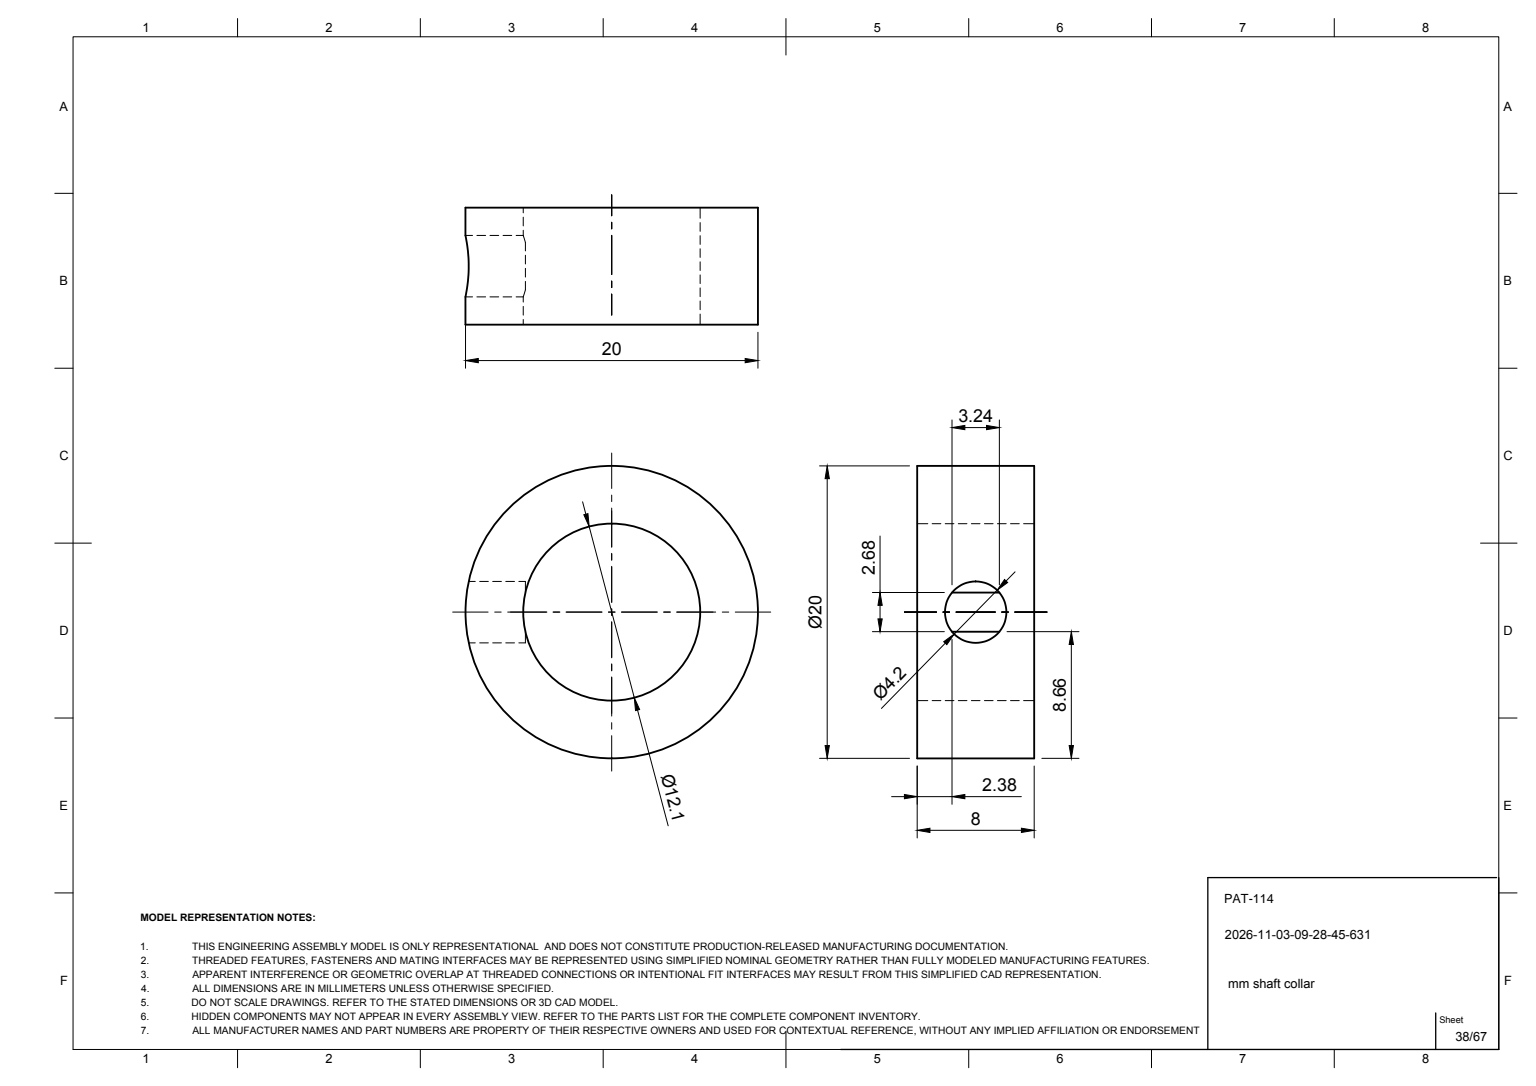
ISO-10303-21;
HEADER;
/* Generated by software containing ST-Developer
 * from STEP Tools, Inc. (www.steptools.com) 
 */

FILE_DESCRIPTION(
/* description */ ('Two-stage gear reducer in split housing'),
/* implementation_level */ '2;1');

FILE_NAME(
/* name */ 'mm shaft collar.step',
/* time_stamp */ '2026-10-28T03:22:31-07:00',
/* author */ (''),
/* organization */ (''),
/* preprocessor_version */ 'ST-DEVELOPER v20.2',
/* originating_system */ 'Autodesk Translation Framework v15.17.0.0',
/* authorisation */ '');

FILE_SCHEMA (('AUTOMOTIVE_DESIGN { 1 0 10303 214 3 1 1 }'));
ENDSEC;

DATA;
#10=MECHANICAL_DESIGN_GEOMETRIC_PRESENTATION_REPRESENTATION('',(#1278),#73366);
#963=B_SPLINE_CURVE_WITH_KNOTS('',3,(#25465,#25466,#25467,#25468,#25469,
#25470,#25471,#25472,#25473,#25474),.UNSPECIFIED.,.F.,.F.,(4,2,2,2,4),(0.818088904349178,
0.878131747417165,0.957937926194036,1.03774410497091,1.09778694803889),
 .UNSPECIFIED.);
#964=B_SPLINE_CURVE_WITH_KNOTS('',3,(#25480,#25481,#25482,#25483,#25484,
#25485,#25486,#25487,#25488,#25489,#25490,#25491,#25492,#25493,#25494,#25495,
#25496,#25497),.UNSPECIFIED.,.F.,.F.,(4,2,2,2,2,2,2,2,4),(0.,0.0793616477694788,
0.158723295538958,0.238079516586307,0.317435737633657,0.396791958681006,
0.476148179728356,0.555509827497835,0.634871475267313),.UNSPECIFIED.);
#965=B_SPLINE_CURVE_WITH_KNOTS('',3,(#25498,#25499,#25500,#25501,#25502,
#25503,#25504,#25505,#25506,#25507,#25508,#25509,#25510,#25511,#25512,#25513,
#25514,#25515),.UNSPECIFIED.,.F.,.F.,(4,2,2,2,2,2,2,2,4),(0.634871475267313,
0.714233123036792,0.793594770806271,0.87295099185362,0.95230721290097,1.03166343394832,
1.11101965499567,1.19038130276515,1.26974295053463),.UNSPECIFIED.);
#966=B_SPLINE_CURVE_WITH_KNOTS('',3,(#25518,#25519,#25520,#25521,#25522,
#25523,#25524,#25525,#25526,#25527),.UNSPECIFIED.,.F.,.F.,(4,2,2,2,4),(0.17946362021982,
0.239506463287808,0.319312642064679,0.39911882084155,0.459161663909537),
 .UNSPECIFIED.);
#1151=SHAPE_REPRESENTATION_RELATIONSHIP('SRR','None',#73641,#1207);
#1207=ADVANCED_BREP_SHAPE_REPRESENTATION('',(#1347),#73337);
#1278=STYLED_ITEM('',(#73988),#1347);
#1347=MANIFOLD_SOLID_BREP('Body1',#16168);
#1539=FACE_BOUND('',#3506,.T.);
#1540=FACE_BOUND('',#3508,.T.);
#1541=FACE_BOUND('',#3510,.T.);
#1542=FACE_BOUND('',#3512,.T.);
#1806=PLANE('',#17779);
#1807=PLANE('',#17784);
#1808=PLANE('',#17791);
#1809=PLANE('',#17792);
#2424=FACE_OUTER_BOUND('',#3502,.T.);
#2425=FACE_OUTER_BOUND('',#3503,.T.);
#2426=FACE_OUTER_BOUND('',#3504,.T.);
#2427=FACE_OUTER_BOUND('',#3505,.T.);
#2428=FACE_OUTER_BOUND('',#3507,.T.);
#2429=FACE_OUTER_BOUND('',#3509,.T.);
#2430=FACE_OUTER_BOUND('',#3511,.T.);
#3502=EDGE_LOOP('',(#12319,#12320));
#3503=EDGE_LOOP('',(#12321,#12322,#12323,#12324,#12325,#12326,#12327,#12328,
#12329));
#3504=EDGE_LOOP('',(#12330,#12331,#12332));
#3505=EDGE_LOOP('',(#12333,#12334,#12335,#12336));
#3506=EDGE_LOOP('',(#12337,#12338,#12339,#12340));
#3507=EDGE_LOOP('',(#12341,#12342,#12343,#12344));
#3508=EDGE_LOOP('',(#12345,#12346));
#3509=EDGE_LOOP('',(#12347));
#3510=EDGE_LOOP('',(#12348));
#3511=EDGE_LOOP('',(#12349));
#3512=EDGE_LOOP('',(#12350));
#4490=LINE('',#25461,#5514);
#4491=LINE('',#25478,#5515);
#4492=LINE('',#25529,#5516);
#4493=LINE('',#25534,#5517);
#4494=LINE('',#25540,#5518);
#5514=VECTOR('',#20828,1.);
#5515=VECTOR('',#20835,0.21);
#5516=VECTOR('',#20840,1.);
#5517=VECTOR('',#20845,0.605);
#5518=VECTOR('',#20852,1.);
#6544=CIRCLE('',#17780,0.21);
#6545=CIRCLE('',#17782,0.21);
#6546=CIRCLE('',#17783,0.21);
#6547=CIRCLE('',#17786,0.605);
#6548=CIRCLE('',#17787,0.605);
#6549=CIRCLE('',#17789,1.);
#6550=CIRCLE('',#17790,1.);
#7443=VERTEX_POINT('',#25459);
#7444=VERTEX_POINT('',#25460);
#7445=VERTEX_POINT('',#25464);
#7446=VERTEX_POINT('',#25475);
#7447=VERTEX_POINT('',#25477);
#7448=VERTEX_POINT('',#25479);
#7449=VERTEX_POINT('',#25516);
#7450=VERTEX_POINT('',#25531);
#7451=VERTEX_POINT('',#25533);
#7452=VERTEX_POINT('',#25537);
#7453=VERTEX_POINT('',#25539);
#9213=EDGE_CURVE('',#7443,#7444,#4490,.T.);
#9214=EDGE_CURVE('',#7443,#7444,#6544,.T.);
#9215=EDGE_CURVE('',#7445,#7443,#963,.T.);
#9216=EDGE_CURVE('',#7446,#7445,#6545,.T.);
#9217=EDGE_CURVE('',#7446,#7447,#4491,.T.);
#9218=EDGE_CURVE('',#7448,#7447,#964,.T.);
#9219=EDGE_CURVE('',#7447,#7448,#965,.T.);
#9220=EDGE_CURVE('',#7449,#7446,#6546,.T.);
#9221=EDGE_CURVE('',#7444,#7449,#966,.T.);
#9222=EDGE_CURVE('',#7449,#7445,#4492,.T.);
#9223=EDGE_CURVE('',#7450,#7450,#6547,.T.);
#9224=EDGE_CURVE('',#7450,#7451,#4493,.T.);
#9225=EDGE_CURVE('',#7451,#7451,#6548,.T.);
#9226=EDGE_CURVE('',#7452,#7452,#6549,.T.);
#9227=EDGE_CURVE('',#7452,#7453,#4494,.T.);
#9228=EDGE_CURVE('',#7453,#7453,#6550,.T.);
#12319=ORIENTED_EDGE('',*,*,#9213,.F.);
#12320=ORIENTED_EDGE('',*,*,#9214,.T.);
#12321=ORIENTED_EDGE('',*,*,#9215,.F.);
#12322=ORIENTED_EDGE('',*,*,#9216,.F.);
#12323=ORIENTED_EDGE('',*,*,#9217,.T.);
#12324=ORIENTED_EDGE('',*,*,#9218,.F.);
#12325=ORIENTED_EDGE('',*,*,#9219,.F.);
#12326=ORIENTED_EDGE('',*,*,#9217,.F.);
#12327=ORIENTED_EDGE('',*,*,#9220,.F.);
#12328=ORIENTED_EDGE('',*,*,#9221,.F.);
#12329=ORIENTED_EDGE('',*,*,#9214,.F.);
#12330=ORIENTED_EDGE('',*,*,#9222,.F.);
#12331=ORIENTED_EDGE('',*,*,#9220,.T.);
#12332=ORIENTED_EDGE('',*,*,#9216,.T.);
#12333=ORIENTED_EDGE('',*,*,#9223,.F.);
#12334=ORIENTED_EDGE('',*,*,#9224,.T.);
#12335=ORIENTED_EDGE('',*,*,#9225,.T.);
#12336=ORIENTED_EDGE('',*,*,#9224,.F.);
#12337=ORIENTED_EDGE('',*,*,#9221,.T.);
#12338=ORIENTED_EDGE('',*,*,#9222,.T.);
#12339=ORIENTED_EDGE('',*,*,#9215,.T.);
#12340=ORIENTED_EDGE('',*,*,#9213,.T.);
#12341=ORIENTED_EDGE('',*,*,#9226,.F.);
#12342=ORIENTED_EDGE('',*,*,#9227,.T.);
#12343=ORIENTED_EDGE('',*,*,#9228,.T.);
#12344=ORIENTED_EDGE('',*,*,#9227,.F.);
#12345=ORIENTED_EDGE('',*,*,#9218,.T.);
#12346=ORIENTED_EDGE('',*,*,#9219,.T.);
#12347=ORIENTED_EDGE('',*,*,#9226,.T.);
#12348=ORIENTED_EDGE('',*,*,#9223,.T.);
#12349=ORIENTED_EDGE('',*,*,#9228,.F.);
#12350=ORIENTED_EDGE('',*,*,#9225,.F.);
#15076=CYLINDRICAL_SURFACE('',#17781,0.21);
#15077=CYLINDRICAL_SURFACE('',#17785,0.605);
#15078=CYLINDRICAL_SURFACE('',#17788,1.);
#15631=ADVANCED_FACE('',(#2424),#1806,.T.);
#15632=ADVANCED_FACE('',(#2425),#15076,.F.);
#15633=ADVANCED_FACE('',(#2426),#1807,.T.);
#15634=ADVANCED_FACE('',(#2427,#1539),#15077,.F.);
#15635=ADVANCED_FACE('',(#2428,#1540),#15078,.T.);
#15636=ADVANCED_FACE('',(#2429,#1541),#1808,.T.);
#15637=ADVANCED_FACE('',(#2430,#1542),#1809,.F.);
#16168=CLOSED_SHELL('',(#15631,#15632,#15633,#15634,#15635,#15636,#15637));
#17778=AXIS2_PLACEMENT_3D('',#25457,#20824,#20825);
#17779=AXIS2_PLACEMENT_3D('',#25458,#20826,#20827);
#17780=AXIS2_PLACEMENT_3D('',#25462,#20829,#20830);
#17781=AXIS2_PLACEMENT_3D('',#25463,#20831,#20832);
#17782=AXIS2_PLACEMENT_3D('',#25476,#20833,#20834);
#17783=AXIS2_PLACEMENT_3D('',#25517,#20836,#20837);
#17784=AXIS2_PLACEMENT_3D('',#25528,#20838,#20839);
#17785=AXIS2_PLACEMENT_3D('',#25530,#20841,#20842);
#17786=AXIS2_PLACEMENT_3D('',#25532,#20843,#20844);
#17787=AXIS2_PLACEMENT_3D('',#25535,#20846,#20847);
#17788=AXIS2_PLACEMENT_3D('',#25536,#20848,#20849);
#17789=AXIS2_PLACEMENT_3D('',#25538,#20850,#20851);
#17790=AXIS2_PLACEMENT_3D('',#25541,#20853,#20854);
#17791=AXIS2_PLACEMENT_3D('',#25542,#20855,#20856);
#17792=AXIS2_PLACEMENT_3D('',#25543,#20857,#20858);
#20824=DIRECTION('axis',(0.,0.,1.));
#20825=DIRECTION('refdir',(1.,0.,0.));
#20826=DIRECTION('center_axis',(0.,0.,1.));
#20827=DIRECTION('ref_axis',(1.,0.,0.));
#20828=DIRECTION('',(0.,1.,0.));
#20829=DIRECTION('center_axis',(0.,0.,1.));
#20830=DIRECTION('ref_axis',(1.,0.,0.));
#20831=DIRECTION('center_axis',(0.,0.,1.));
#20832=DIRECTION('ref_axis',(1.,0.,0.));
#20833=DIRECTION('center_axis',(0.,0.,1.));
#20834=DIRECTION('ref_axis',(1.,0.,0.));
#20835=DIRECTION('',(0.,0.,1.));
#20836=DIRECTION('center_axis',(0.,0.,1.));
#20837=DIRECTION('ref_axis',(1.,0.,0.));
#20838=DIRECTION('center_axis',(0.,0.,1.));
#20839=DIRECTION('ref_axis',(1.,0.,0.));
#20840=DIRECTION('',(0.,-1.,0.));
#20841=DIRECTION('center_axis',(0.,1.,0.));
#20842=DIRECTION('ref_axis',(1.,0.,0.));
#20843=DIRECTION('center_axis',(0.,-1.,0.));
#20844=DIRECTION('ref_axis',(1.,0.,0.));
#20845=DIRECTION('',(0.,-1.,0.));
#20846=DIRECTION('center_axis',(0.,-1.,0.));
#20847=DIRECTION('ref_axis',(1.,0.,0.));
#20848=DIRECTION('center_axis',(0.,1.,0.));
#20849=DIRECTION('ref_axis',(1.,0.,0.));
#20850=DIRECTION('center_axis',(0.,1.,0.));
#20851=DIRECTION('ref_axis',(1.,0.,0.));
#20852=DIRECTION('',(0.,-1.,0.));
#20853=DIRECTION('center_axis',(0.,1.,0.));
#20854=DIRECTION('ref_axis',(1.,0.,0.));
#20855=DIRECTION('center_axis',(0.,1.,0.));
#20856=DIRECTION('ref_axis',(1.,0.,0.));
#20857=DIRECTION('center_axis',(0.,1.,0.));
#20858=DIRECTION('ref_axis',(1.,0.,0.));
#25457=CARTESIAN_POINT('',(0.,0.,0.));
#25458=CARTESIAN_POINT('Origin',(0.,-8.2,10.59));
#25459=CARTESIAN_POINT('',(0.133884278389952,-8.36178689687364,10.59));
#25460=CARTESIAN_POINT('',(0.133884278389952,-8.03821310312636,10.59));
#25461=CARTESIAN_POINT('',(0.133884278389952,-8.6,10.59));
#25462=CARTESIAN_POINT('Origin',(0.,-8.2,10.59));
#25463=CARTESIAN_POINT('Origin',(0.,-8.2,10.59));
#25464=CARTESIAN_POINT('',(-0.133884278389952,-8.36178689687364,10.59));
#25465=CARTESIAN_POINT('Ctrl Pts',(-0.133884278389951,-8.36178689687364,
10.59));
#25466=CARTESIAN_POINT('Ctrl Pts',(-0.118254395260798,-8.37472116821763,
10.5935467722442));
#25467=CARTESIAN_POINT('Ctrl Pts',(-0.100109787682296,-8.38579931658744,
10.5969822478996));
#25468=CARTESIAN_POINT('Ctrl Pts',(-0.0548298721325181,-8.40463856105443,
10.6030741628997));
#25469=CARTESIAN_POINT('Ctrl Pts',(-0.0266020595922904,-8.41,10.605));
#25470=CARTESIAN_POINT('Ctrl Pts',(0.0266020595922903,-8.41,10.605));
#25471=CARTESIAN_POINT('Ctrl Pts',(0.0548298721325192,-8.40463856105443,
10.6030741628997));
#25472=CARTESIAN_POINT('Ctrl Pts',(0.100109787682297,-8.38579931658744,
10.5969822478996));
#25473=CARTESIAN_POINT('Ctrl Pts',(0.118254395260798,-8.37472116821763,
10.5935467722442));
#25474=CARTESIAN_POINT('Ctrl Pts',(0.133884278389951,-8.36178689687364,
10.59));
#25475=CARTESIAN_POINT('',(-0.21,-8.2,10.59));
#25476=CARTESIAN_POINT('Origin',(0.,-8.2,10.59));
#25477=CARTESIAN_POINT('',(-0.21,-8.2,10.9777013859047));
#25478=CARTESIAN_POINT('',(-0.21,-8.2,10.59));
#25479=CARTESIAN_POINT('',(0.21,-8.2,10.9777013859047));
#25480=CARTESIAN_POINT('Ctrl Pts',(0.21,-8.2,10.9777013859047));
#25481=CARTESIAN_POINT('Ctrl Pts',(0.21,-8.22645388258983,10.9777013859047));
#25482=CARTESIAN_POINT('Ctrl Pts',(0.204697017125528,-8.25461525830868,
10.9788864661322));
#25483=CARTESIAN_POINT('Ctrl Pts',(0.18324175151553,-8.30633042130174,10.9831286999115));
#25484=CARTESIAN_POINT('Ctrl Pts',(0.167093586802906,-8.32989126129544,
10.9861204479665));
#25485=CARTESIAN_POINT('Ctrl Pts',(0.129892533236543,-8.36709231486181,
10.9917064515638));
#25486=CARTESIAN_POINT('Ctrl Pts',(0.106331154992713,-8.38324147510569,
10.994669144466));
#25487=CARTESIAN_POINT('Ctrl Pts',(0.0546141143983528,-8.40469746372443,
10.9988444923724));
#25488=CARTESIAN_POINT('Ctrl Pts',(0.0264520736824499,-8.41,11.));
#25489=CARTESIAN_POINT('Ctrl Pts',(-0.0264520736824498,-8.41,11.));
#25490=CARTESIAN_POINT('Ctrl Pts',(-0.0546141143983527,-8.40469746372443,
10.9988444923724));
#25491=CARTESIAN_POINT('Ctrl Pts',(-0.106331154992713,-8.38324147510569,
10.994669144466));
#25492=CARTESIAN_POINT('Ctrl Pts',(-0.129892533236543,-8.36709231486181,
10.9917064515638));
#25493=CARTESIAN_POINT('Ctrl Pts',(-0.167093586802906,-8.32989126129544,
10.9861204479665));
#25494=CARTESIAN_POINT('Ctrl Pts',(-0.18324175151553,-8.30633042130174,
10.9831286999115));
#25495=CARTESIAN_POINT('Ctrl Pts',(-0.204697017125528,-8.25461525830868,
10.9788864661322));
#25496=CARTESIAN_POINT('Ctrl Pts',(-0.21,-8.22645388258983,10.9777013859047));
#25497=CARTESIAN_POINT('Ctrl Pts',(-0.21,-8.2,10.9777013859047));
#25498=CARTESIAN_POINT('Ctrl Pts',(-0.21,-8.2,10.9777013859047));
#25499=CARTESIAN_POINT('Ctrl Pts',(-0.21,-8.17354611741017,10.9777013859047));
#25500=CARTESIAN_POINT('Ctrl Pts',(-0.204697017125528,-8.14538474169131,
10.9788864661322));
#25501=CARTESIAN_POINT('Ctrl Pts',(-0.18324175151553,-8.09366957869826,
10.9831286999115));
#25502=CARTESIAN_POINT('Ctrl Pts',(-0.167093586802907,-8.07010873870455,
10.9861204479665));
#25503=CARTESIAN_POINT('Ctrl Pts',(-0.129892533236543,-8.03290768513819,
10.9917064515638));
#25504=CARTESIAN_POINT('Ctrl Pts',(-0.106331154992713,-8.01675852489431,
10.994669144466));
#25505=CARTESIAN_POINT('Ctrl Pts',(-0.0546141143983529,-7.99530253627557,
10.9988444923724));
#25506=CARTESIAN_POINT('Ctrl Pts',(-0.0264520736824499,-7.99,11.));
#25507=CARTESIAN_POINT('Ctrl Pts',(0.0264520736824497,-7.99,11.));
#25508=CARTESIAN_POINT('Ctrl Pts',(0.0546141143983529,-7.99530253627557,
10.9988444923724));
#25509=CARTESIAN_POINT('Ctrl Pts',(0.106331154992714,-8.01675852489431,
10.994669144466));
#25510=CARTESIAN_POINT('Ctrl Pts',(0.129892533236543,-8.03290768513819,
10.9917064515638));
#25511=CARTESIAN_POINT('Ctrl Pts',(0.167093586802906,-8.07010873870455,
10.9861204479665));
#25512=CARTESIAN_POINT('Ctrl Pts',(0.18324175151553,-8.09366957869826,10.9831286999115));
#25513=CARTESIAN_POINT('Ctrl Pts',(0.204697017125528,-8.14538474169131,
10.9788864661322));
#25514=CARTESIAN_POINT('Ctrl Pts',(0.21,-8.17354611741017,10.9777013859047));
#25515=CARTESIAN_POINT('Ctrl Pts',(0.21,-8.2,10.9777013859047));
#25516=CARTESIAN_POINT('',(-0.133884278389952,-8.03821310312636,10.59));
#25517=CARTESIAN_POINT('Origin',(0.,-8.2,10.59));
#25518=CARTESIAN_POINT('Ctrl Pts',(0.133884278389952,-8.03821310312636,
10.59));
#25519=CARTESIAN_POINT('Ctrl Pts',(0.118254395260798,-8.02527883178237,
10.5935467722442));
#25520=CARTESIAN_POINT('Ctrl Pts',(0.100109787682297,-8.01420068341256,
10.5969822478996));
#25521=CARTESIAN_POINT('Ctrl Pts',(0.0548298721325187,-7.99536143894557,
10.6030741628997));
#25522=CARTESIAN_POINT('Ctrl Pts',(0.0266020595922903,-7.99,10.605));
#25523=CARTESIAN_POINT('Ctrl Pts',(-0.0266020595922903,-7.99,10.605));
#25524=CARTESIAN_POINT('Ctrl Pts',(-0.0548298721325201,-7.99536143894557,
10.6030741628997));
#25525=CARTESIAN_POINT('Ctrl Pts',(-0.100109787682298,-8.01420068341256,
10.5969822478996));
#25526=CARTESIAN_POINT('Ctrl Pts',(-0.118254395260797,-8.02527883178237,
10.5935467722442));
#25527=CARTESIAN_POINT('Ctrl Pts',(-0.133884278389951,-8.03821310312636,
10.59));
#25528=CARTESIAN_POINT('Origin',(0.,-8.2,10.59));
#25529=CARTESIAN_POINT('',(-0.133884278389952,-8.6,10.59));
#25530=CARTESIAN_POINT('Origin',(0.,-8.6,10.));
#25531=CARTESIAN_POINT('',(-0.605,-7.8,10.));
#25532=CARTESIAN_POINT('Origin',(0.,-7.8,10.));
#25533=CARTESIAN_POINT('',(-0.605,-8.6,10.));
#25534=CARTESIAN_POINT('',(-0.605,-8.6,10.));
#25535=CARTESIAN_POINT('Origin',(0.,-8.6,10.));
#25536=CARTESIAN_POINT('Origin',(0.,-8.6,10.));
#25537=CARTESIAN_POINT('',(-1.,-7.8,10.));
#25538=CARTESIAN_POINT('Origin',(0.,-7.8,10.));
#25539=CARTESIAN_POINT('',(-1.,-8.6,10.));
#25540=CARTESIAN_POINT('',(-1.,-8.6,10.));
#25541=CARTESIAN_POINT('Origin',(0.,-8.6,10.));
#25542=CARTESIAN_POINT('Origin',(0.,-7.8,10.));
#25543=CARTESIAN_POINT('Origin',(0.,-8.6,10.));
#73273=UNCERTAINTY_MEASURE_WITH_UNIT(LENGTH_MEASURE(0.001),#73367,
'DISTANCE_ACCURACY_VALUE',
'Maximum model space distance between geometric entities at asserted c
onnectivities');
#73302=UNCERTAINTY_MEASURE_WITH_UNIT(LENGTH_MEASURE(0.001),#73367,
'DISTANCE_ACCURACY_VALUE',
'Maximum model space distance between geometric entities at asserted c
onnectivities');
#73337=(
GEOMETRIC_REPRESENTATION_CONTEXT(3)
GLOBAL_UNCERTAINTY_ASSIGNED_CONTEXT((#73273))
GLOBAL_UNIT_ASSIGNED_CONTEXT((#73367,#73369,#73370))
REPRESENTATION_CONTEXT('','3D')
);
#73366=(
GEOMETRIC_REPRESENTATION_CONTEXT(3)
GLOBAL_UNCERTAINTY_ASSIGNED_CONTEXT((#73302))
GLOBAL_UNIT_ASSIGNED_CONTEXT((#73367,#73369,#73370))
REPRESENTATION_CONTEXT('','3D')
);
#73367=(
LENGTH_UNIT()
NAMED_UNIT(*)
SI_UNIT(.CENTI.,.METRE.)
);
#73369=(
NAMED_UNIT(*)
PLANE_ANGLE_UNIT()
SI_UNIT($,.RADIAN.)
);
#73370=(
NAMED_UNIT(*)
SI_UNIT($,.STERADIAN.)
SOLID_ANGLE_UNIT()
);
#73405=SHAPE_DEFINITION_REPRESENTATION(#73538,#73641);
#73538=PRODUCT_DEFINITION_SHAPE('',$,#73705);
#73641=SHAPE_REPRESENTATION('',(#17778),#73337);
#73670=PRODUCT_DEFINITION_CONTEXT('part definition',#73861,'design');
#73705=PRODUCT_DEFINITION('mm shaft collar','mm shaft collar',#73768,#73670);
#73768=PRODUCT_DEFINITION_FORMATION('',$,#73897);
#73861=APPLICATION_CONTEXT(
'Core Data for Automotive Mechanical Design Process');
#73862=PRODUCT_CONTEXT('part definition',#73861,'mechanical');
#73897=PRODUCT('mm shaft collar','mm shaft collar','mm shaft collar',(#73862));
#73982=COLOUR_RGB('Grey',0.48,0.52,0.57);
#73983=FILL_AREA_STYLE_COLOUR('',#73982);
#73984=FILL_AREA_STYLE('',(#73983));
#73985=SURFACE_STYLE_FILL_AREA(#73984);
#73986=SURFACE_SIDE_STYLE('',(#73985));
#73987=SURFACE_STYLE_USAGE(.BOTH.,#73986);
#73988=PRESENTATION_STYLE_ASSIGNMENT((#73987));
ENDSEC;
END-ISO-10303-21;
